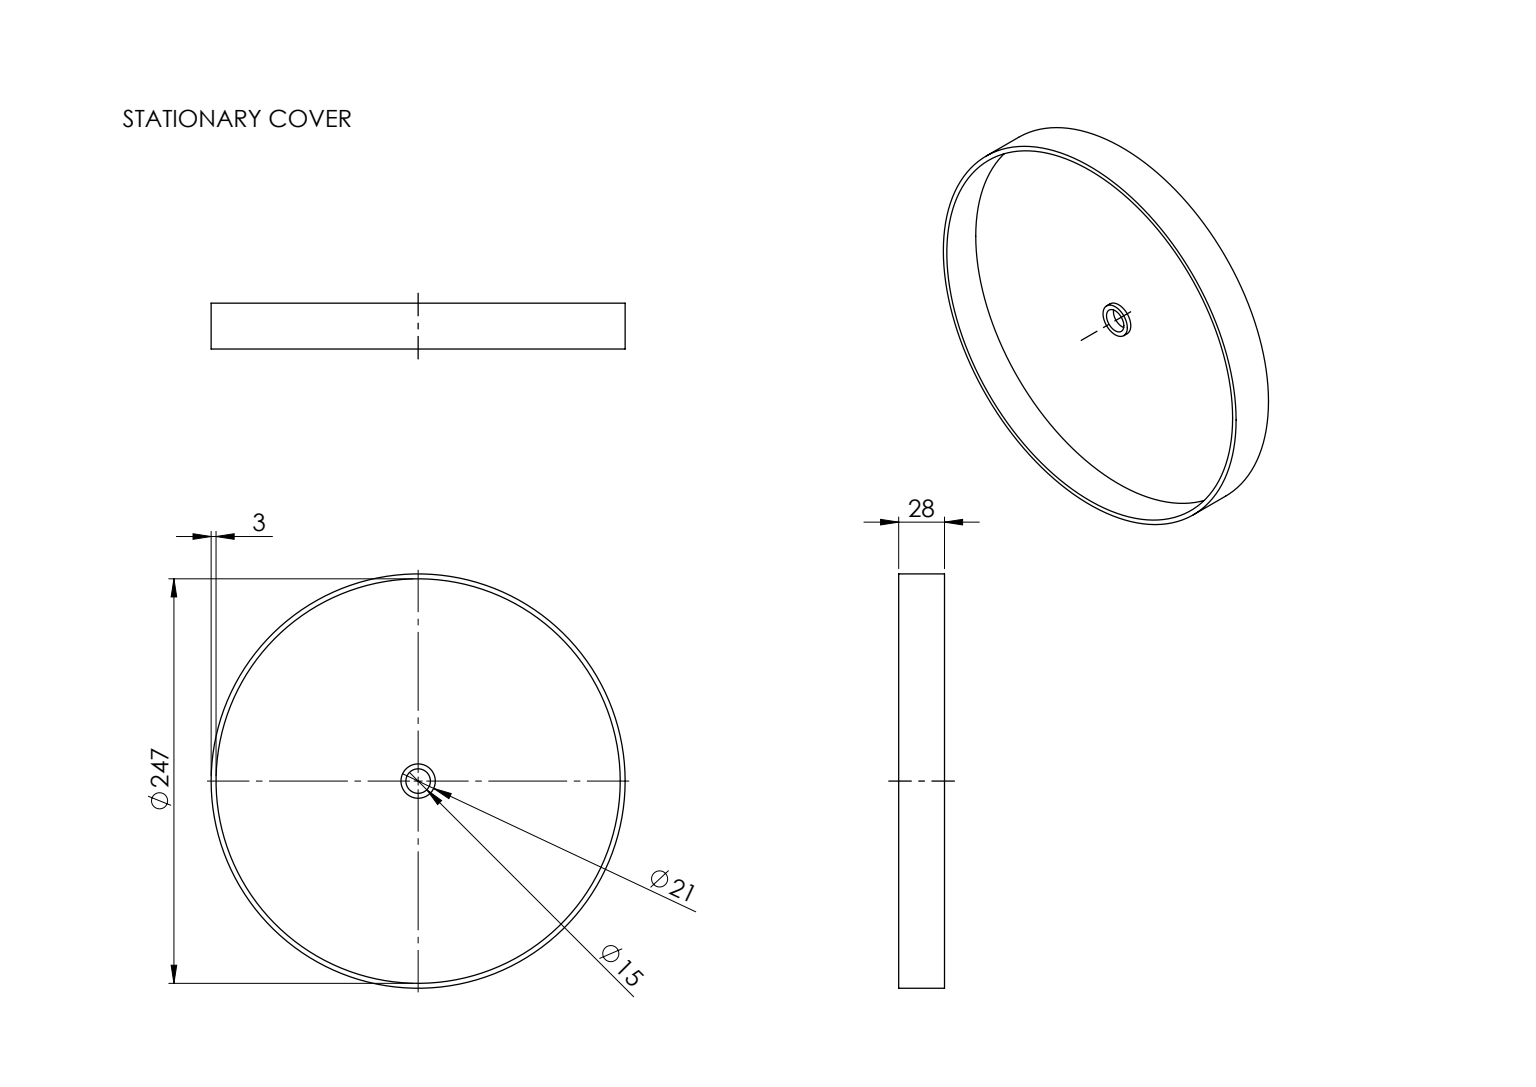
ISO-10303-21;
HEADER;
FILE_DESCRIPTION (('STEP AP214'),
    '1' );
FILE_NAME ('stationary cover.step',
    '2026-09-30T13:58:28',
    ( '' ),
    ( '' ),
    'SwSTEP 2.0',
    'SolidWorks 2026',
    '' );
FILE_SCHEMA (( 'AUTOMOTIVE_DESIGN' ));
ENDSEC;

DATA;
#19=ORIENTED_EDGE ( 'NONE', *, *, #690, .T. ) ;
#139=PLANE ( 'NONE',  #5077 ) ;
#149=CARTESIAN_POINT ( 'NONE',  ( 126.5000000000000000, 0.000000000000000000, -3.000000000000000000 ) ) ;
#174=VECTOR ( 'NONE', #10367, 1000.000000000000000 ) ;
#208=VECTOR ( 'NONE', #9875, 1000.000000000000000 ) ;
#299=ORIENTED_EDGE ( 'NONE', *, *, #7580, .F. ) ;
#364=DIRECTION ( 'NONE',  ( 0.000000000000000000, 0.000000000000000000, 1.000000000000000000 ) ) ;
#374=VERTEX_POINT ( 'NONE', #17387 ) ;
#381=PRODUCT_DEFINITION ( 'UNKNOWN', '', #13101, #3862 ) ;
#524=EDGE_CURVE ( 'NONE', #12679, #374, #13850, .T. ) ;
#537=DIRECTION ( 'NONE',  ( 0.000000000000000000, 0.000000000000000000, 1.000000000000000000 ) ) ;
#566=ORIENTED_EDGE ( 'NONE', *, *, #12735, .T. ) ;
#602=DIRECTION ( 'NONE',  ( -1.000000000000000000, 0.000000000000000000, 0.000000000000000000 ) ) ;
#660=DIRECTION ( 'NONE',  ( -0.000000000000000000, -0.000000000000000000, -1.000000000000000000 ) ) ;
#690=EDGE_CURVE ( 'NONE', #13273, #6116, #14924, .T. ) ;
#710=DIRECTION ( 'NONE',  ( -1.000000000000000000, 0.000000000000000000, 0.000000000000000000 ) ) ;
#780=CYLINDRICAL_SURFACE ( 'NONE', #12998, 10.49999999999999822 ) ;
#854=ORIENTED_EDGE ( 'NONE', *, *, #12020, .F. ) ;
#896=ORIENTED_EDGE ( 'NONE', *, *, #17448, .T. ) ;
#916=CARTESIAN_POINT ( 'NONE',  ( 126.5000000000000000, 0.000000000000000000, -3.000000000000000000 ) ) ;
#1011=CARTESIAN_POINT ( 'NONE',  ( 7.500000000000000000, 9.184850993605147944E-16, 3.000000000000000000 ) ) ;
#1076=FACE_OUTER_BOUND ( 'NONE', #15687, .T. ) ;
#1098=ORIENTED_EDGE ( 'NONE', *, *, #9059, .T. ) ;
#1238=FACE_OUTER_BOUND ( 'NONE', #7650, .T. ) ;
#1247=LINE ( 'NONE', #9295, #5456 ) ;
#1274=CIRCLE ( 'NONE', #16070, 126.5000000000000000 ) ;
#1450=ORIENTED_EDGE ( 'NONE', *, *, #2028, .T. ) ;
#1558=VERTEX_POINT ( 'NONE', #916 ) ;
#1618=EDGE_CURVE ( 'NONE', #3657, #11363, #3460, .T. ) ;
#1654=EDGE_CURVE ( 'NONE', #2973, #3104, #5936, .T. ) ;
#1845=CARTESIAN_POINT ( 'NONE',  ( -126.5000000000000000, 1.549178200921401833E-14, -3.000000000000000000 ) ) ;
#1879=FACE_OUTER_BOUND ( 'NONE', #11836, .T. ) ;
#1889=VERTEX_POINT ( 'NONE', #18919 ) ;
#2028=EDGE_CURVE ( 'NONE', #14712, #2259, #15451, .T. ) ;
#2108=COLOUR_RGB ( '', 0.66274510, 0.83137255, 0.94901961) ;
#2237=( LENGTH_UNIT ( ) NAMED_UNIT ( * ) SI_UNIT ( .MILLI., .METRE. ) );
#2259=VERTEX_POINT ( 'NONE', #3725 ) ;
#2263=EDGE_CURVE ( 'NONE', #13273, #3104, #7147, .T. ) ;
#2315=CYLINDRICAL_SURFACE ( 'NONE', #18232, 10.49999999999999822 ) ;
#2321=DIRECTION ( 'NONE',  ( 0.000000000000000000, 0.000000000000000000, 1.000000000000000000 ) ) ;
#2322=ORIENTED_EDGE ( 'NONE', *, *, #1654, .F. ) ;
#2341=ORIENTED_EDGE ( 'NONE', *, *, #1654, .T. ) ;
#2377=CIRCLE ( 'NONE', #7329, 7.500000000000000000 ) ;
#2390=ORIENTED_EDGE ( 'NONE', *, *, #18284, .T. ) ;
#2492=CIRCLE ( 'NONE', #10954, 10.49999999999999822 ) ;
#2614=AXIS2_PLACEMENT_3D ( 'NONE', #21710, #6595, #20064 ) ;
#2713=ADVANCED_FACE ( 'NONE', ( #6919 ), #19057, .F. ) ;
#2783=AXIS2_PLACEMENT_3D ( 'NONE', #3915, #8564, #3697 ) ;
#2806=DIRECTION ( 'NONE',  ( -1.000000000000000000, 0.000000000000000000, 0.000000000000000000 ) ) ;
#2863=DIRECTION ( 'NONE',  ( 1.000000000000000000, 0.000000000000000000, 0.000000000000000000 ) ) ;
#2973=VERTEX_POINT ( 'NONE', #3023 ) ;
#3023=CARTESIAN_POINT ( 'NONE',  ( 10.49999999999999822, 1.285879139104720633E-15, 0.000000000000000000 ) ) ;
#3065=CIRCLE ( 'NONE', #4834, 126.5000000000000000 ) ;
#3075=ADVANCED_FACE ( 'NONE', ( #21684, #6574 ), #6687, .F. ) ;
#3104=VERTEX_POINT ( 'NONE', #20148 ) ;
#3191=AXIS2_PLACEMENT_3D ( 'NONE', #7977, #19251, #6006 ) ;
#3257=DIRECTION ( 'NONE',  ( 0.000000000000000000, 0.000000000000000000, 1.000000000000000000 ) ) ;
#3275=ORIENTED_EDGE ( 'NONE', *, *, #12162, .T. ) ;
#3460=CIRCLE ( 'NONE', #21448, 123.5000000000000142 ) ;
#3464=CYLINDRICAL_SURFACE ( 'NONE', #4166, 123.5000000000000142 ) ;
#3527=CARTESIAN_POINT ( 'NONE',  ( 0.000000000000000000, 0.000000000000000000, 0.000000000000000000 ) ) ;
#3642=AXIS2_PLACEMENT_3D ( 'NONE', #6737, #4626, #6623 ) ;
#3657=VERTEX_POINT ( 'NONE', #13912 ) ;
#3697=DIRECTION ( 'NONE',  ( -1.000000000000000000, 0.000000000000000000, 0.000000000000000000 ) ) ;
#3725=CARTESIAN_POINT ( 'NONE',  ( -7.500000000000000000, 0.000000000000000000, 3.000000000000000000 ) ) ;
#3855=AXIS2_PLACEMENT_3D ( 'NONE', #17877, #6284, #6057 ) ;
#3862=PRODUCT_DEFINITION_CONTEXT ( 'detailed design', #13334, 'design' ) ;
#3870=MECHANICAL_DESIGN_GEOMETRIC_PRESENTATION_REPRESENTATION('',(#17280),#5626);
#3883=DIRECTION ( 'NONE',  ( 1.000000000000000000, 0.000000000000000000, 0.000000000000000000 ) ) ;
#3892=ORIENTED_EDGE ( 'NONE', *, *, #21618, .F. ) ;
#3900=SURFACE_STYLE_USAGE ( .BOTH. , #17284 ) ;
#3915=CARTESIAN_POINT ( 'NONE',  ( 0.000000000000000000, 0.000000000000000000, 3.000000000000000000 ) ) ;
#4097=ORIENTED_EDGE ( 'NONE', *, *, #11338, .F. ) ;
#4166=AXIS2_PLACEMENT_3D ( 'NONE', #6789, #16950, #7005 ) ;
#4309=DIRECTION ( 'NONE',  ( 1.000000000000000000, 0.000000000000000000, 0.000000000000000000 ) ) ;
#4387=PLANE ( 'NONE',  #3855 ) ;
#4473=FILL_AREA_STYLE_COLOUR ( '', #2108 ) ;
#4553=FACE_BOUND ( 'NONE', #10873, .T. ) ;
#4626=DIRECTION ( 'NONE',  ( 0.000000000000000000, 0.000000000000000000, 1.000000000000000000 ) ) ;
#4684=CARTESIAN_POINT ( 'NONE',  ( 10.49999999999999822, 1.285879139104720633E-15, 3.000000000000000000 ) ) ;
#4714=ORIENTED_EDGE ( 'NONE', *, *, #10117, .F. ) ;
#4733=CIRCLE ( 'NONE', #2614, 10.49999999999999822 ) ;
#4834=AXIS2_PLACEMENT_3D ( 'NONE', #19659, #19539, #2863 ) ;
#4838=ORIENTED_EDGE ( 'NONE', *, *, #20951, .F. ) ;
#4846=DIRECTION ( 'NONE',  ( 0.000000000000000000, 0.000000000000000000, 1.000000000000000000 ) ) ;
#4994=ORIENTED_EDGE ( 'NONE', *, *, #1618, .F. ) ;
#5077=AXIS2_PLACEMENT_3D ( 'NONE', #13615, #364, #20368 ) ;
#5353=( GEOMETRIC_REPRESENTATION_CONTEXT ( 3 ) GLOBAL_UNCERTAINTY_ASSIGNED_CONTEXT ( ( #18892 ) ) GLOBAL_UNIT_ASSIGNED_CONTEXT ( ( #14064, #12395, #20487 ) ) REPRESENTATION_CONTEXT ( 'NONE', 'WORKASPACE' ) );
#5411=UNCERTAINTY_MEASURE_WITH_UNIT (LENGTH_MEASURE( 1.000000000000000082E-05 ), #2237, 'distance_accuracy_value', 'NONE');
#5456=VECTOR ( 'NONE', #21467, 1000.000000000000000 ) ;
#5606=CARTESIAN_POINT ( 'NONE',  ( -10.49999999999999822, 0.000000000000000000, 3.000000000000000000 ) ) ;
#5626=( GEOMETRIC_REPRESENTATION_CONTEXT ( 3 ) GLOBAL_UNCERTAINTY_ASSIGNED_CONTEXT ( ( #19835 ) ) GLOBAL_UNIT_ASSIGNED_CONTEXT ( ( #9316, #21376, #10986 ) ) REPRESENTATION_CONTEXT ( 'NONE', 'WORKASPACE' ) );
#5632=DIRECTION ( 'NONE',  ( 0.000000000000000000, 0.000000000000000000, 1.000000000000000000 ) ) ;
#5670=FILL_AREA_STYLE ('',( #10852 ) ) ;
#5717=LINE ( 'NONE', #20852, #7248 ) ;
#5789=CARTESIAN_POINT ( 'NONE',  ( 0.000000000000000000, 0.000000000000000000, 0.000000000000000000 ) ) ;
#5870=CIRCLE ( 'NONE', #18223, 123.5000000000000142 ) ;
#5931=AXIS2_PLACEMENT_3D ( 'NONE', #20889, #12710, #4309 ) ;
#5936=CIRCLE ( 'NONE', #18638, 10.49999999999999822 ) ;
#5937=DIRECTION ( 'NONE',  ( 0.000000000000000000, 0.000000000000000000, 1.000000000000000000 ) ) ;
#6000=DIRECTION ( 'NONE',  ( -1.000000000000000000, 0.000000000000000000, 0.000000000000000000 ) ) ;
#6003=SHAPE_REPRESENTATION ( 'stationary cover', ( #15567 ), #9570 ) ;
#6006=DIRECTION ( 'NONE',  ( 1.000000000000000000, 0.000000000000000000, 0.000000000000000000 ) ) ;
#6008=VECTOR ( 'NONE', #14948, 1000.000000000000000 ) ;
#6033=FILL_AREA_STYLE ('',( #4473 ) ) ;
#6057=DIRECTION ( 'NONE',  ( 1.000000000000000000, 0.000000000000000000, -0.000000000000000000 ) ) ;
#6070=COLOUR_RGB ( '', 0.66274510, 0.83137255, 0.94901961) ;
#6116=VERTEX_POINT ( 'NONE', #9571 ) ;
#6123=DIRECTION ( 'NONE',  ( -0.000000000000000000, -0.000000000000000000, 1.000000000000000000 ) ) ;
#6147=EDGE_LOOP ( 'NONE', ( #3275, #8389 ) ) ;
#6170=CYLINDRICAL_SURFACE ( 'NONE', #8848, 123.5000000000000142 ) ;
#6222=EDGE_CURVE ( 'NONE', #2259, #14712, #14585, .T. ) ;
#6284=DIRECTION ( 'NONE',  ( 0.000000000000000000, 0.000000000000000000, 1.000000000000000000 ) ) ;
#6368=LINE ( 'NONE', #4684, #208 ) ;
#6437=ADVANCED_BREP_SHAPE_REPRESENTATION ( '', ( #20833, #15567 ), #9570 ) ;
#6566=CARTESIAN_POINT ( 'NONE',  ( -7.500000000000000000, 0.000000000000000000, 3.000000000000000000 ) ) ;
#6574=FACE_OUTER_BOUND ( 'NONE', #19364, .T. ) ;
#6595=DIRECTION ( 'NONE',  ( -0.000000000000000000, -0.000000000000000000, 1.000000000000000000 ) ) ;
#6623=DIRECTION ( 'NONE',  ( 1.000000000000000000, 0.000000000000000000, 0.000000000000000000 ) ) ;
#6687=PLANE ( 'NONE',  #8328 ) ;
#6726=CARTESIAN_POINT ( 'NONE',  ( 0.000000000000000000, 0.000000000000000000, -3.000000000000000000 ) ) ;
#6737=CARTESIAN_POINT ( 'NONE',  ( 0.000000000000000000, 0.000000000000000000, 3.000000000000000000 ) ) ;
#6747=PLANE ( 'NONE',  #7360 ) ;
#6750=EDGE_CURVE ( 'NONE', #3104, #2973, #4733, .T. ) ;
#6768=ORIENTED_EDGE ( 'NONE', *, *, #1618, .T. ) ;
#6789=CARTESIAN_POINT ( 'NONE',  ( 0.000000000000000000, 0.000000000000000000, -3.000000000000000000 ) ) ;
#6919=FACE_OUTER_BOUND ( 'NONE', #11533, .T. ) ;
#7005=DIRECTION ( 'NONE',  ( 1.000000000000000000, 0.000000000000000000, 0.000000000000000000 ) ) ;
#7040=DIRECTION ( 'NONE',  ( 0.000000000000000000, 0.000000000000000000, 1.000000000000000000 ) ) ;
#7118=VERTEX_POINT ( 'NONE', #8613 ) ;
#7147=LINE ( 'NONE', #5606, #12571 ) ;
#7195=ORIENTED_EDGE ( 'NONE', *, *, #20951, .T. ) ;
#7248=VECTOR ( 'NONE', #5937, 1000.000000000000000 ) ;
#7278=ORIENTED_EDGE ( 'NONE', *, *, #16211, .T. ) ;
#7290=CARTESIAN_POINT ( 'NONE',  ( 7.500000000000000000, 9.184850993605147944E-16, -3.000000000000000000 ) ) ;
#7329=AXIS2_PLACEMENT_3D ( 'NONE', #19277, #9209, #16179 ) ;
#7360=AXIS2_PLACEMENT_3D ( 'NONE', #3527, #11393, #20210 ) ;
#7409=DIRECTION ( 'NONE',  ( -1.000000000000000000, 0.000000000000000000, 0.000000000000000000 ) ) ;
#7441=SHAPE_REPRESENTATION_RELATIONSHIP ( 'NONE' , 'NONE' ,  #6003, #6437 ) ;
#7444=ORIENTED_EDGE ( 'NONE', *, *, #19727, .F. ) ;
#7504=VECTOR ( 'NONE', #4846, 1000.000000000000000 ) ;
#7552=CYLINDRICAL_SURFACE ( 'NONE', #7894, 126.5000000000000000 ) ;
#7580=EDGE_CURVE ( 'NONE', #3657, #21386, #18661, .T. ) ;
#7650=EDGE_LOOP ( 'NONE', ( #7856, #566, #7195, #9460 ) ) ;
#7663=DIRECTION ( 'NONE',  ( -1.000000000000000000, 0.000000000000000000, 0.000000000000000000 ) ) ;
#7712=DIRECTION ( 'NONE',  ( 1.000000000000000000, 0.000000000000000000, 0.000000000000000000 ) ) ;
#7818=CARTESIAN_POINT ( 'NONE',  ( 0.000000000000000000, 0.000000000000000000, 25.00000000000000000 ) ) ;
#7856=ORIENTED_EDGE ( 'NONE', *, *, #8934, .F. ) ;
#7880=AXIS2_PLACEMENT_3D ( 'NONE', #13969, #12517, #602 ) ;
#7894=AXIS2_PLACEMENT_3D ( 'NONE', #9101, #12631, #15618 ) ;
#7977=CARTESIAN_POINT ( 'NONE',  ( 0.000000000000000000, 0.000000000000000000, -3.000000000000000000 ) ) ;
#8024=CARTESIAN_POINT ( 'NONE',  ( -126.5000000000000000, 1.549178200921401833E-14, 25.00000000000000000 ) ) ;
#8091=EDGE_LOOP ( 'NONE', ( #20759, #854 ) ) ;
#8110=DIRECTION ( 'NONE',  ( 1.000000000000000000, 0.000000000000000000, -0.000000000000000000 ) ) ;
#8173=ORIENTED_EDGE ( 'NONE', *, *, #6222, .F. ) ;
#8328=AXIS2_PLACEMENT_3D ( 'NONE', #13402, #13497, #8110 ) ;
#8389=ORIENTED_EDGE ( 'NONE', *, *, #524, .T. ) ;
#8536=FACE_OUTER_BOUND ( 'NONE', #6147, .T. ) ;
#8543=FACE_OUTER_BOUND ( 'NONE', #12394, .T. ) ;
#8564=DIRECTION ( 'NONE',  ( -0.000000000000000000, -0.000000000000000000, -1.000000000000000000 ) ) ;
#8613=CARTESIAN_POINT ( 'NONE',  ( -7.500000000000000000, 0.000000000000000000, -3.000000000000000000 ) ) ;
#8848=AXIS2_PLACEMENT_3D ( 'NONE', #6726, #7040, #14987 ) ;
#8867=( NAMED_UNIT ( * ) SI_UNIT ( $, .STERADIAN. ) SOLID_ANGLE_UNIT ( ) );
#8869=ORIENTED_EDGE ( 'NONE', *, *, #6750, .T. ) ;
#8879=CARTESIAN_POINT ( 'NONE',  ( 0.000000000000000000, 0.000000000000000000, 3.000000000000000000 ) ) ;
#8934=EDGE_CURVE ( 'NONE', #9557, #12679, #1247, .T. ) ;
#8938=EDGE_CURVE ( 'NONE', #7118, #9088, #17801, .T. ) ;
#9059=EDGE_CURVE ( 'NONE', #2259, #7118, #21677, .T. ) ;
#9063=DIRECTION ( 'NONE',  ( 0.000000000000000000, 0.000000000000000000, 1.000000000000000000 ) ) ;
#9088=VERTEX_POINT ( 'NONE', #7290 ) ;
#9101=CARTESIAN_POINT ( 'NONE',  ( 0.000000000000000000, 0.000000000000000000, -3.000000000000000000 ) ) ;
#9209=DIRECTION ( 'NONE',  ( -0.000000000000000000, -0.000000000000000000, -1.000000000000000000 ) ) ;
#9241=ORIENTED_EDGE ( 'NONE', *, *, #7580, .T. ) ;
#9295=CARTESIAN_POINT ( 'NONE',  ( -126.5000000000000000, 1.549178200921401833E-14, -3.000000000000000000 ) ) ;
#9316=( LENGTH_UNIT ( ) NAMED_UNIT ( * ) SI_UNIT ( .MILLI., .METRE. ) );
#9460=ORIENTED_EDGE ( 'NONE', *, *, #524, .F. ) ;
#9557=VERTEX_POINT ( 'NONE', #1845 ) ;
#9570=( GEOMETRIC_REPRESENTATION_CONTEXT ( 3 ) GLOBAL_UNCERTAINTY_ASSIGNED_CONTEXT ( ( #5411 ) ) GLOBAL_UNIT_ASSIGNED_CONTEXT ( ( #2237, #17381, #8867 ) ) REPRESENTATION_CONTEXT ( 'NONE', 'WORKASPACE' ) );
#9571=CARTESIAN_POINT ( 'NONE',  ( 10.49999999999999822, 1.285879139104720633E-15, 3.000000000000000000 ) ) ;
#9619=ORIENTED_EDGE ( 'NONE', *, *, #6750, .F. ) ;
#9748=EDGE_LOOP ( 'NONE', ( #16670, #11074 ) ) ;
#9846=ORIENTED_EDGE ( 'NONE', *, *, #16532, .F. ) ;
#9875=DIRECTION ( 'NONE',  ( -0.000000000000000000, -0.000000000000000000, -1.000000000000000000 ) ) ;
#10015=AXIS2_PLACEMENT_3D ( 'NONE', #8879, #20821, #710 ) ;
#10070=CLOSED_SHELL ( 'NONE', ( #2713, #14730, #11357, #21751, #18490, #21316, #3075, #11678, #18818, #20531, #17338, #11384 ) ) ;
#10117=EDGE_CURVE ( 'NONE', #14712, #9088, #10537, .T. ) ;
#10263=EDGE_LOOP ( 'NONE', ( #6768, #20126 ) ) ;
#10367=DIRECTION ( 'NONE',  ( -0.000000000000000000, -0.000000000000000000, -1.000000000000000000 ) ) ;
#10494=CARTESIAN_POINT ( 'NONE',  ( 0.000000000000000000, 0.000000000000000000, 3.000000000000000000 ) ) ;
#10537=LINE ( 'NONE', #10860, #19217 ) ;
#10578=ORIENTED_EDGE ( 'NONE', *, *, #2028, .F. ) ;
#10590=CARTESIAN_POINT ( 'NONE',  ( 0.000000000000000000, 0.000000000000000000, 25.00000000000000000 ) ) ;
#10632=EDGE_LOOP ( 'NONE', ( #8173, #10578 ) ) ;
#10671=DIRECTION ( 'NONE',  ( -0.000000000000000000, -0.000000000000000000, -1.000000000000000000 ) ) ;
#10798=ORIENTED_EDGE ( 'NONE', *, *, #9059, .F. ) ;
#10852=FILL_AREA_STYLE_COLOUR ( '', #6070 ) ;
#10860=CARTESIAN_POINT ( 'NONE',  ( 7.500000000000000000, 9.184850993605147944E-16, 3.000000000000000000 ) ) ;
#10861=DIRECTION ( 'NONE',  ( -0.000000000000000000, -0.000000000000000000, 1.000000000000000000 ) ) ;
#10873=EDGE_LOOP ( 'NONE', ( #9619, #2322 ) ) ;
#10954=AXIS2_PLACEMENT_3D ( 'NONE', #12374, #2321, #7712 ) ;
#10986=( NAMED_UNIT ( * ) SI_UNIT ( $, .STERADIAN. ) SOLID_ANGLE_UNIT ( ) );
#11061=ORIENTED_EDGE ( 'NONE', *, *, #8938, .T. ) ;
#11074=ORIENTED_EDGE ( 'NONE', *, *, #18284, .F. ) ;
#11096=PRESENTATION_STYLE_ASSIGNMENT (( #17958 ) ) ;
#11130=FACE_BOUND ( 'NONE', #10632, .T. ) ;
#11338=EDGE_CURVE ( 'NONE', #11363, #3657, #14572, .T. ) ;
#11357=ADVANCED_FACE ( 'NONE', ( #21036 ), #7552, .T. ) ;
#11363=VERTEX_POINT ( 'NONE', #16054 ) ;
#11384=ADVANCED_FACE ( 'NONE', ( #15737 ), #19381, .F. ) ;
#11393=DIRECTION ( 'NONE',  ( 0.000000000000000000, 0.000000000000000000, -1.000000000000000000 ) ) ;
#11533=EDGE_LOOP ( 'NONE', ( #18231, #15251, #2390, #10798 ) ) ;
#11678=ADVANCED_FACE ( 'NONE', ( #8536, #15262 ), #139, .T. ) ;
#11747=LINE ( 'NONE', #149, #6008 ) ;
#11757=EDGE_LOOP ( 'NONE', ( #896, #12419, #16814, #4838 ) ) ;
#11836=EDGE_LOOP ( 'NONE', ( #7444, #12752, #20510, #8869 ) ) ;
#12020=EDGE_CURVE ( 'NONE', #1889, #21386, #5870, .T. ) ;
#12070=APPLICATION_CONTEXT ( 'automotive_design' ) ;
#12159=AXIS2_PLACEMENT_3D ( 'NONE', #7818, #19855, #18212 ) ;
#12162=EDGE_CURVE ( 'NONE', #374, #12679, #14986, .T. ) ;
#12374=CARTESIAN_POINT ( 'NONE',  ( 0.000000000000000000, 0.000000000000000000, 3.000000000000000000 ) ) ;
#12387=FACE_OUTER_BOUND ( 'NONE', #16263, .T. ) ;
#12394=EDGE_LOOP ( 'NONE', ( #9846, #4994, #9241, #7278 ) ) ;
#12395=( NAMED_UNIT ( * ) PLANE_ANGLE_UNIT ( ) SI_UNIT ( $, .RADIAN. ) );
#12419=ORIENTED_EDGE ( 'NONE', *, *, #8934, .T. ) ;
#12517=DIRECTION ( 'NONE',  ( -0.000000000000000000, -0.000000000000000000, 1.000000000000000000 ) ) ;
#12571=VECTOR ( 'NONE', #10671, 1000.000000000000000 ) ;
#12603=CARTESIAN_POINT ( 'NONE',  ( 0.000000000000000000, 0.000000000000000000, 3.000000000000000000 ) ) ;
#12624=DIRECTION ( 'NONE',  ( -0.000000000000000000, -0.000000000000000000, -1.000000000000000000 ) ) ;
#12631=DIRECTION ( 'NONE',  ( 0.000000000000000000, 0.000000000000000000, 1.000000000000000000 ) ) ;
#12640=SURFACE_SIDE_STYLE ('',( #14742 ) ) ;
#12679=VERTEX_POINT ( 'NONE', #8024 ) ;
#12710=DIRECTION ( 'NONE',  ( 0.000000000000000000, 0.000000000000000000, 1.000000000000000000 ) ) ;
#12735=EDGE_CURVE ( 'NONE', #9557, #1558, #1274, .T. ) ;
#12752=ORIENTED_EDGE ( 'NONE', *, *, #690, .F. ) ;
#12837=DIRECTION ( 'NONE',  ( -0.000000000000000000, -0.000000000000000000, -1.000000000000000000 ) ) ;
#12998=AXIS2_PLACEMENT_3D ( 'NONE', #12603, #19352, #6000 ) ;
#13101=PRODUCT_DEFINITION_FORMATION_WITH_SPECIFIED_SOURCE ( 'ANY', '', #18865, .NOT_KNOWN. ) ;
#13230=CARTESIAN_POINT ( 'NONE',  ( 123.5000000000000142, 0.000000000000000000, -3.000000000000000000 ) ) ;
#13273=VERTEX_POINT ( 'NONE', #15261 ) ;
#13334=APPLICATION_CONTEXT ( 'automotive_design' ) ;
#13402=CARTESIAN_POINT ( 'NONE',  ( 0.000000000000000000, 0.000000000000000000, -3.000000000000000000 ) ) ;
#13497=DIRECTION ( 'NONE',  ( 0.000000000000000000, 0.000000000000000000, 1.000000000000000000 ) ) ;
#13573=FACE_OUTER_BOUND ( 'NONE', #10263, .T. ) ;
#13615=CARTESIAN_POINT ( 'NONE',  ( 0.000000000000000000, 0.000000000000000000, 25.00000000000000000 ) ) ;
#13745=PRESENTATION_STYLE_ASSIGNMENT (( #3900 ) ) ;
#13850=CIRCLE ( 'NONE', #14560, 126.5000000000000000 ) ;
#13912=CARTESIAN_POINT ( 'NONE',  ( 123.5000000000000142, 0.000000000000000000, 0.000000000000000000 ) ) ;
#13955=SURFACE_STYLE_FILL_AREA ( #5670 ) ;
#13969=CARTESIAN_POINT ( 'NONE',  ( 0.000000000000000000, 0.000000000000000000, 0.000000000000000000 ) ) ;
#14064=( LENGTH_UNIT ( ) NAMED_UNIT ( * ) SI_UNIT ( .MILLI., .METRE. ) );
#14222=ORIENTED_EDGE ( 'NONE', *, *, #19727, .T. ) ;
#14392=ORIENTED_EDGE ( 'NONE', *, *, #2263, .F. ) ;
#14498=CYLINDRICAL_SURFACE ( 'NONE', #3191, 126.5000000000000000 ) ;
#14506=CARTESIAN_POINT ( 'NONE',  ( 0.000000000000000000, 0.000000000000000000, -3.000000000000000000 ) ) ;
#14560=AXIS2_PLACEMENT_3D ( 'NONE', #16577, #14912, #21762 ) ;
#14572=CIRCLE ( 'NONE', #7880, 123.5000000000000142 ) ;
#14585=CIRCLE ( 'NONE', #3642, 7.500000000000000000 ) ;
#14712=VERTEX_POINT ( 'NONE', #1011 ) ;
#14720=ORIENTED_EDGE ( 'NONE', *, *, #21618, .T. ) ;
#14730=ADVANCED_FACE ( 'NONE', ( #12387 ), #780, .T. ) ;
#14742=SURFACE_STYLE_FILL_AREA ( #6033 ) ;
#14778=FACE_OUTER_BOUND ( 'NONE', #18728, .T. ) ;
#14912=DIRECTION ( 'NONE',  ( 0.000000000000000000, 0.000000000000000000, 1.000000000000000000 ) ) ;
#14924=CIRCLE ( 'NONE', #16688, 10.49999999999999822 ) ;
#14948=DIRECTION ( 'NONE',  ( 0.000000000000000000, 0.000000000000000000, 1.000000000000000000 ) ) ;
#14965=CARTESIAN_POINT ( 'NONE',  ( 0.000000000000000000, 0.000000000000000000, -3.000000000000000000 ) ) ;
#14986=CIRCLE ( 'NONE', #12159, 126.5000000000000000 ) ;
#14987=DIRECTION ( 'NONE',  ( 1.000000000000000000, 0.000000000000000000, 0.000000000000000000 ) ) ;
#15244=CARTESIAN_POINT ( 'NONE',  ( 123.5000000000000142, 0.000000000000000000, 25.00000000000000000 ) ) ;
#15251=ORIENTED_EDGE ( 'NONE', *, *, #10117, .T. ) ;
#15261=CARTESIAN_POINT ( 'NONE',  ( -10.49999999999999822, 0.000000000000000000, 3.000000000000000000 ) ) ;
#15262=FACE_BOUND ( 'NONE', #8091, .T. ) ;
#15341=CIRCLE ( 'NONE', #17809, 123.5000000000000142 ) ;
#15451=CIRCLE ( 'NONE', #5931, 7.500000000000000000 ) ;
#15567=AXIS2_PLACEMENT_3D ( 'NONE', #21837, #20187, #17085 ) ;
#15584=ORIENTED_EDGE ( 'NONE', *, *, #12735, .F. ) ;
#15618=DIRECTION ( 'NONE',  ( 1.000000000000000000, 0.000000000000000000, 0.000000000000000000 ) ) ;
#15671=CARTESIAN_POINT ( 'NONE',  ( 0.000000000000000000, 0.000000000000000000, 3.000000000000000000 ) ) ;
#15687=EDGE_LOOP ( 'NONE', ( #4097, #18966, #20242, #299 ) ) ;
#15737=FACE_OUTER_BOUND ( 'NONE', #19470, .T. ) ;
#16054=CARTESIAN_POINT ( 'NONE',  ( -123.5000000000000142, 1.512438796946981289E-14, 0.000000000000000000 ) ) ;
#16070=AXIS2_PLACEMENT_3D ( 'NONE', #14965, #3257, #16410 ) ;
#16179=DIRECTION ( 'NONE',  ( 1.000000000000000000, 0.000000000000000000, 0.000000000000000000 ) ) ;
#16211=EDGE_CURVE ( 'NONE', #21386, #1889, #15341, .T. ) ;
#16263=EDGE_LOOP ( 'NONE', ( #3892, #14222, #2341, #14392 ) ) ;
#16270=DIRECTION ( 'NONE',  ( 1.000000000000000000, 0.000000000000000000, 0.000000000000000000 ) ) ;
#16410=DIRECTION ( 'NONE',  ( 1.000000000000000000, 0.000000000000000000, 0.000000000000000000 ) ) ;
#16532=EDGE_CURVE ( 'NONE', #11363, #1889, #5717, .T. ) ;
#16559=PRODUCT_DEFINITION_SHAPE ( 'NONE', 'NONE',  #381 ) ;
#16577=CARTESIAN_POINT ( 'NONE',  ( 0.000000000000000000, 0.000000000000000000, 25.00000000000000000 ) ) ;
#16670=ORIENTED_EDGE ( 'NONE', *, *, #8938, .F. ) ;
#16688=AXIS2_PLACEMENT_3D ( 'NONE', #15671, #5632, #19104 ) ;
#16814=ORIENTED_EDGE ( 'NONE', *, *, #12162, .F. ) ;
#16950=DIRECTION ( 'NONE',  ( 0.000000000000000000, 0.000000000000000000, 1.000000000000000000 ) ) ;
#17085=DIRECTION ( 'NONE',  ( 1.000000000000000000, 0.000000000000000000, 0.000000000000000000 ) ) ;
#17280=STYLED_ITEM ( 'NONE', ( #11096 ), #20833 ) ;
#17284=SURFACE_SIDE_STYLE ('',( #13955 ) ) ;
#17338=ADVANCED_FACE ( 'NONE', ( #1879 ), #2315, .T. ) ;
#17381=( NAMED_UNIT ( * ) PLANE_ANGLE_UNIT ( ) SI_UNIT ( $, .RADIAN. ) );
#17387=CARTESIAN_POINT ( 'NONE',  ( 126.5000000000000000, 0.000000000000000000, 25.00000000000000000 ) ) ;
#17448=EDGE_CURVE ( 'NONE', #1558, #9557, #3065, .T. ) ;
#17801=CIRCLE ( 'NONE', #20286, 7.500000000000000000 ) ;
#17809=AXIS2_PLACEMENT_3D ( 'NONE', #19124, #9063, #3883 ) ;
#17877=CARTESIAN_POINT ( 'NONE',  ( 0.000000000000000000, 0.000000000000000000, 3.000000000000000000 ) ) ;
#17958=SURFACE_STYLE_USAGE ( .BOTH. , #12640 ) ;
#18151=SHAPE_DEFINITION_REPRESENTATION ( #16559, #6003 ) ;
#18212=DIRECTION ( 'NONE',  ( 1.000000000000000000, 0.000000000000000000, 0.000000000000000000 ) ) ;
#18223=AXIS2_PLACEMENT_3D ( 'NONE', #10590, #537, #21193 ) ;
#18231=ORIENTED_EDGE ( 'NONE', *, *, #6222, .T. ) ;
#18232=AXIS2_PLACEMENT_3D ( 'NONE', #10494, #660, #7409 ) ;
#18284=EDGE_CURVE ( 'NONE', #9088, #7118, #2377, .T. ) ;
#18422=MECHANICAL_DESIGN_GEOMETRIC_PRESENTATION_REPRESENTATION('',(#20866),#5353);
#18490=ADVANCED_FACE ( 'NONE', ( #8543 ), #3464, .F. ) ;
#18638=AXIS2_PLACEMENT_3D ( 'NONE', #21251, #6123, #2806 ) ;
#18661=LINE ( 'NONE', #13230, #7504 ) ;
#18728=EDGE_LOOP ( 'NONE', ( #19, #14720 ) ) ;
#18818=ADVANCED_FACE ( 'NONE', ( #4553, #13573 ), #6747, .F. ) ;
#18865=PRODUCT ( 'stationary cover', 'stationary cover', '', ( #19366 ) ) ;
#18892=UNCERTAINTY_MEASURE_WITH_UNIT (LENGTH_MEASURE( 1.000000000000000082E-05 ), #14064, 'distance_accuracy_value', 'NONE');
#18919=CARTESIAN_POINT ( 'NONE',  ( -123.5000000000000142, 1.512438796946981289E-14, 25.00000000000000000 ) ) ;
#18966=ORIENTED_EDGE ( 'NONE', *, *, #16532, .T. ) ;
#19057=CYLINDRICAL_SURFACE ( 'NONE', #2783, 7.500000000000000000 ) ;
#19104=DIRECTION ( 'NONE',  ( 1.000000000000000000, 0.000000000000000000, 0.000000000000000000 ) ) ;
#19124=CARTESIAN_POINT ( 'NONE',  ( 0.000000000000000000, 0.000000000000000000, 25.00000000000000000 ) ) ;
#19217=VECTOR ( 'NONE', #12624, 1000.000000000000000 ) ;
#19251=DIRECTION ( 'NONE',  ( 0.000000000000000000, 0.000000000000000000, 1.000000000000000000 ) ) ;
#19277=CARTESIAN_POINT ( 'NONE',  ( 0.000000000000000000, 0.000000000000000000, -3.000000000000000000 ) ) ;
#19352=DIRECTION ( 'NONE',  ( -0.000000000000000000, -0.000000000000000000, -1.000000000000000000 ) ) ;
#19364=EDGE_LOOP ( 'NONE', ( #21485, #15584 ) ) ;
#19366=PRODUCT_CONTEXT ( 'NONE', #12070, 'mechanical' ) ;
#19381=CYLINDRICAL_SURFACE ( 'NONE', #10015, 7.500000000000000000 ) ;
#19470=EDGE_LOOP ( 'NONE', ( #4714, #1450, #1098, #11061 ) ) ;
#19539=DIRECTION ( 'NONE',  ( 0.000000000000000000, 0.000000000000000000, 1.000000000000000000 ) ) ;
#19659=CARTESIAN_POINT ( 'NONE',  ( 0.000000000000000000, 0.000000000000000000, -3.000000000000000000 ) ) ;
#19727=EDGE_CURVE ( 'NONE', #6116, #2973, #6368, .T. ) ;
#19835=UNCERTAINTY_MEASURE_WITH_UNIT (LENGTH_MEASURE( 1.000000000000000082E-05 ), #9316, 'distance_accuracy_value', 'NONE');
#19855=DIRECTION ( 'NONE',  ( 0.000000000000000000, 0.000000000000000000, 1.000000000000000000 ) ) ;
#20064=DIRECTION ( 'NONE',  ( -1.000000000000000000, 0.000000000000000000, 0.000000000000000000 ) ) ;
#20126=ORIENTED_EDGE ( 'NONE', *, *, #11338, .T. ) ;
#20148=CARTESIAN_POINT ( 'NONE',  ( -10.49999999999999822, 0.000000000000000000, 0.000000000000000000 ) ) ;
#20187=DIRECTION ( 'NONE',  ( 0.000000000000000000, 0.000000000000000000, 1.000000000000000000 ) ) ;
#20210=DIRECTION ( 'NONE',  ( -1.000000000000000000, 0.000000000000000000, -0.000000000000000000 ) ) ;
#20242=ORIENTED_EDGE ( 'NONE', *, *, #12020, .T. ) ;
#20286=AXIS2_PLACEMENT_3D ( 'NONE', #14506, #12837, #16270 ) ;
#20368=DIRECTION ( 'NONE',  ( 1.000000000000000000, 0.000000000000000000, -0.000000000000000000 ) ) ;
#20487=( NAMED_UNIT ( * ) SI_UNIT ( $, .STERADIAN. ) SOLID_ANGLE_UNIT ( ) );
#20510=ORIENTED_EDGE ( 'NONE', *, *, #2263, .T. ) ;
#20531=ADVANCED_FACE ( 'NONE', ( #14778, #11130 ), #4387, .T. ) ;
#20759=ORIENTED_EDGE ( 'NONE', *, *, #16211, .F. ) ;
#20821=DIRECTION ( 'NONE',  ( -0.000000000000000000, -0.000000000000000000, -1.000000000000000000 ) ) ;
#20833=MANIFOLD_SOLID_BREP ( 'Cut-Extrude1', #10070 ) ;
#20852=CARTESIAN_POINT ( 'NONE',  ( -123.5000000000000142, 1.512438796946981289E-14, -3.000000000000000000 ) ) ;
#20866=STYLED_ITEM ( 'NONE', ( #13745 ), #6437 ) ;
#20889=CARTESIAN_POINT ( 'NONE',  ( 0.000000000000000000, 0.000000000000000000, 3.000000000000000000 ) ) ;
#20951=EDGE_CURVE ( 'NONE', #1558, #374, #11747, .T. ) ;
#21036=FACE_OUTER_BOUND ( 'NONE', #11757, .T. ) ;
#21193=DIRECTION ( 'NONE',  ( 1.000000000000000000, 0.000000000000000000, 0.000000000000000000 ) ) ;
#21251=CARTESIAN_POINT ( 'NONE',  ( 0.000000000000000000, 0.000000000000000000, 0.000000000000000000 ) ) ;
#21316=ADVANCED_FACE ( 'NONE', ( #1238 ), #14498, .T. ) ;
#21376=( NAMED_UNIT ( * ) PLANE_ANGLE_UNIT ( ) SI_UNIT ( $, .RADIAN. ) );
#21386=VERTEX_POINT ( 'NONE', #15244 ) ;
#21448=AXIS2_PLACEMENT_3D ( 'NONE', #5789, #10861, #7663 ) ;
#21467=DIRECTION ( 'NONE',  ( 0.000000000000000000, 0.000000000000000000, 1.000000000000000000 ) ) ;
#21485=ORIENTED_EDGE ( 'NONE', *, *, #17448, .F. ) ;
#21618=EDGE_CURVE ( 'NONE', #6116, #13273, #2492, .T. ) ;
#21677=LINE ( 'NONE', #6566, #174 ) ;
#21684=FACE_BOUND ( 'NONE', #9748, .T. ) ;
#21710=CARTESIAN_POINT ( 'NONE',  ( 0.000000000000000000, 0.000000000000000000, 0.000000000000000000 ) ) ;
#21751=ADVANCED_FACE ( 'NONE', ( #1076 ), #6170, .F. ) ;
#21762=DIRECTION ( 'NONE',  ( 1.000000000000000000, 0.000000000000000000, 0.000000000000000000 ) ) ;
#21837=CARTESIAN_POINT ( 'NONE',  ( 0.000000000000000000, 0.000000000000000000, 0.000000000000000000 ) ) ;
ENDSEC;
END-ISO-10303-21;
